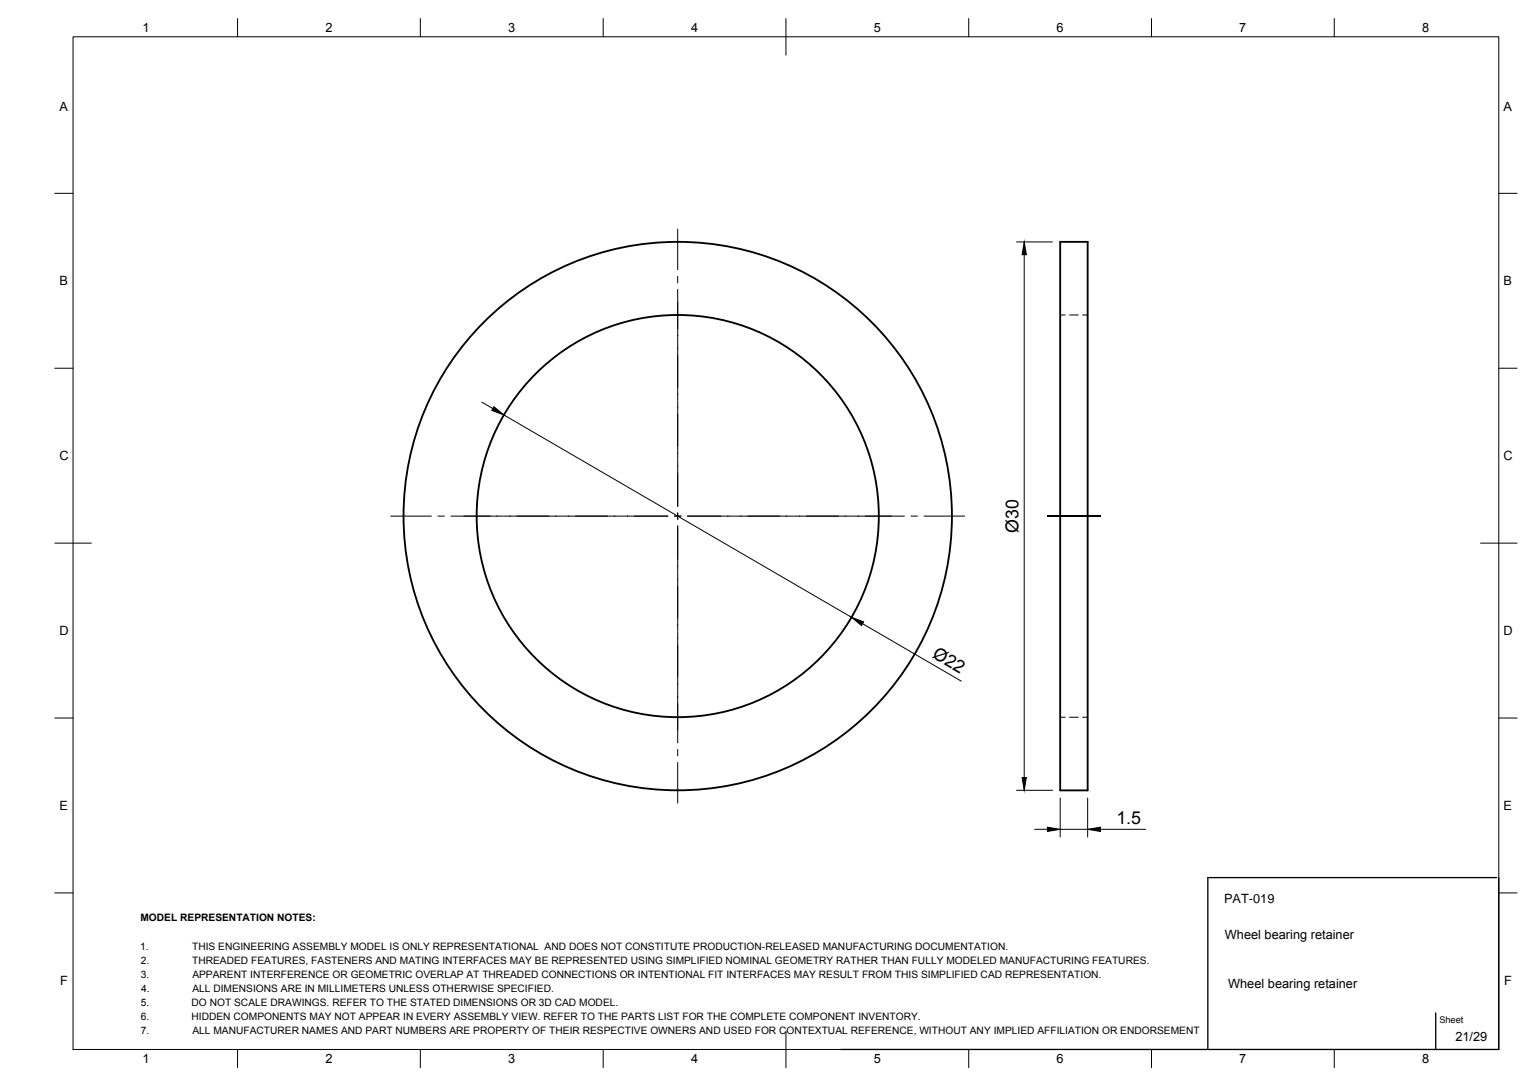
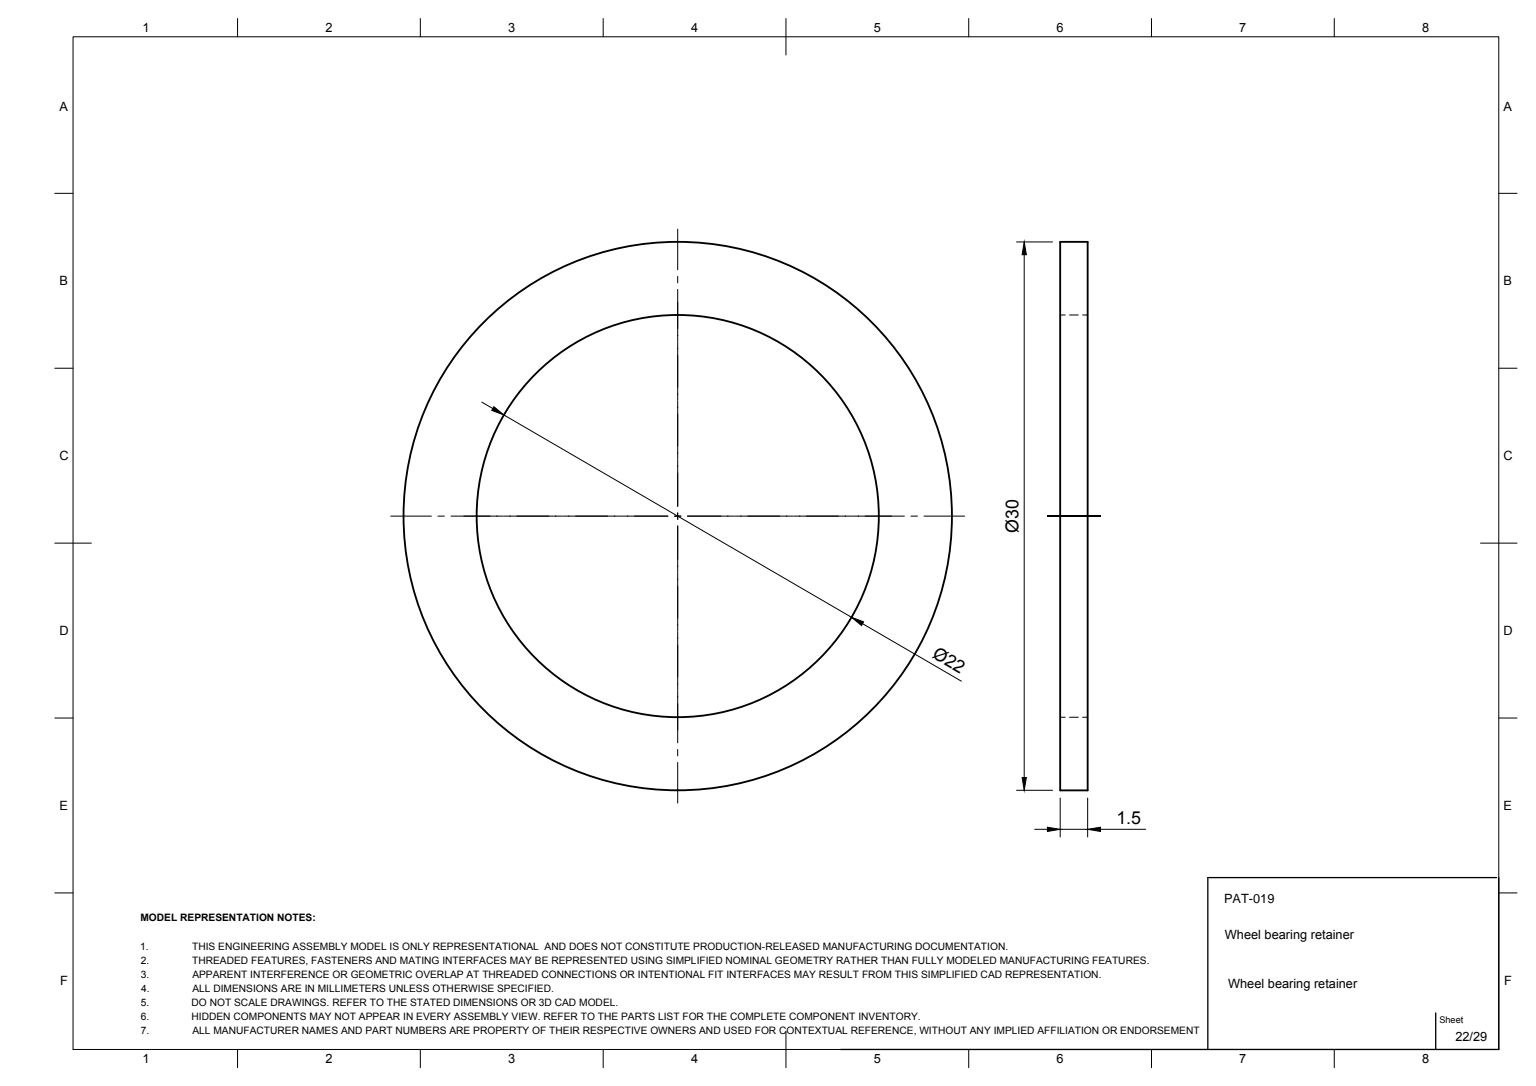
ISO-10303-21;
HEADER;
/* Generated by software containing ST-Developer
 * from STEP Tools, Inc. (www.steptools.com) 
 */

FILE_DESCRIPTION(
/* description */ ('Caster wheel assembly'),
/* implementation_level */ '2;1');

FILE_NAME(
/* name */ 'Wheel bearing retainer.step',
/* time_stamp */ '2026-10-28T03:23:56-07:00',
/* author */ (''),
/* organization */ (''),
/* preprocessor_version */ 'ST-DEVELOPER v20.2',
/* originating_system */ 'Autodesk Translation Framework v15.17.0.0',
/* authorisation */ '');

FILE_SCHEMA (('AUTOMOTIVE_DESIGN { 1 0 10303 214 3 1 1 }'));
ENDSEC;

DATA;
#10=MECHANICAL_DESIGN_GEOMETRIC_PRESENTATION_REPRESENTATION('',(#237),#5385);
#193=SHAPE_REPRESENTATION_RELATIONSHIP('SRR','None',#5490,#215);
#215=ADVANCED_BREP_SHAPE_REPRESENTATION('',(#266),#5377);
#237=STYLED_ITEM('',(#5672),#266);
#266=MANIFOLD_SOLID_BREP('Body1',#2665);
#320=FACE_BOUND('',#740,.T.);
#321=FACE_BOUND('',#742,.T.);
#400=PLANE('',#3151);
#401=PLANE('',#3152);
#530=FACE_OUTER_BOUND('',#737,.T.);
#531=FACE_OUTER_BOUND('',#738,.T.);
#532=FACE_OUTER_BOUND('',#739,.T.);
#533=FACE_OUTER_BOUND('',#741,.T.);
#737=EDGE_LOOP('',(#2192,#2193,#2194,#2195));
#738=EDGE_LOOP('',(#2196,#2197,#2198,#2199));
#739=EDGE_LOOP('',(#2200));
#740=EDGE_LOOP('',(#2201));
#741=EDGE_LOOP('',(#2202));
#742=EDGE_LOOP('',(#2203));
#923=LINE('',#4711,#1057);
#924=LINE('',#4717,#1058);
#1057=VECTOR('',#3866,1.1);
#1058=VECTOR('',#3873,1.5);
#1156=CIRCLE('',#3146,1.1);
#1157=CIRCLE('',#3147,1.1);
#1158=CIRCLE('',#3149,1.5);
#1159=CIRCLE('',#3150,1.5);
#1371=VERTEX_POINT('',#4708);
#1372=VERTEX_POINT('',#4710);
#1373=VERTEX_POINT('',#4714);
#1374=VERTEX_POINT('',#4716);
#1664=EDGE_CURVE('',#1371,#1371,#1156,.T.);
#1665=EDGE_CURVE('',#1371,#1372,#923,.T.);
#1666=EDGE_CURVE('',#1372,#1372,#1157,.T.);
#1667=EDGE_CURVE('',#1373,#1373,#1158,.T.);
#1668=EDGE_CURVE('',#1373,#1374,#924,.T.);
#1669=EDGE_CURVE('',#1374,#1374,#1159,.T.);
#2192=ORIENTED_EDGE('',*,*,#1664,.F.);
#2193=ORIENTED_EDGE('',*,*,#1665,.T.);
#2194=ORIENTED_EDGE('',*,*,#1666,.T.);
#2195=ORIENTED_EDGE('',*,*,#1665,.F.);
#2196=ORIENTED_EDGE('',*,*,#1667,.F.);
#2197=ORIENTED_EDGE('',*,*,#1668,.T.);
#2198=ORIENTED_EDGE('',*,*,#1669,.T.);
#2199=ORIENTED_EDGE('',*,*,#1668,.F.);
#2200=ORIENTED_EDGE('',*,*,#1667,.T.);
#2201=ORIENTED_EDGE('',*,*,#1664,.T.);
#2202=ORIENTED_EDGE('',*,*,#1669,.F.);
#2203=ORIENTED_EDGE('',*,*,#1666,.F.);
#2465=CYLINDRICAL_SURFACE('',#3145,1.1);
#2466=CYLINDRICAL_SURFACE('',#3148,1.5);
#2590=ADVANCED_FACE('',(#530),#2465,.F.);
#2591=ADVANCED_FACE('',(#531),#2466,.T.);
#2592=ADVANCED_FACE('',(#532,#320),#400,.T.);
#2593=ADVANCED_FACE('',(#533,#321),#401,.F.);
#2665=CLOSED_SHELL('',(#2590,#2591,#2592,#2593));
#3144=AXIS2_PLACEMENT_3D('',#4706,#3860,#3861);
#3145=AXIS2_PLACEMENT_3D('',#4707,#3862,#3863);
#3146=AXIS2_PLACEMENT_3D('',#4709,#3864,#3865);
#3147=AXIS2_PLACEMENT_3D('',#4712,#3867,#3868);
#3148=AXIS2_PLACEMENT_3D('',#4713,#3869,#3870);
#3149=AXIS2_PLACEMENT_3D('',#4715,#3871,#3872);
#3150=AXIS2_PLACEMENT_3D('',#4718,#3874,#3875);
#3151=AXIS2_PLACEMENT_3D('',#4719,#3876,#3877);
#3152=AXIS2_PLACEMENT_3D('',#4720,#3878,#3879);
#3860=DIRECTION('axis',(0.,0.,1.));
#3861=DIRECTION('refdir',(1.,0.,0.));
#3862=DIRECTION('center_axis',(0.,1.,0.));
#3863=DIRECTION('ref_axis',(1.,0.,0.));
#3864=DIRECTION('center_axis',(0.,-1.,0.));
#3865=DIRECTION('ref_axis',(1.,0.,0.));
#3866=DIRECTION('',(0.,-1.,0.));
#3867=DIRECTION('center_axis',(0.,-1.,0.));
#3868=DIRECTION('ref_axis',(1.,0.,0.));
#3869=DIRECTION('center_axis',(0.,1.,0.));
#3870=DIRECTION('ref_axis',(1.,0.,0.));
#3871=DIRECTION('center_axis',(0.,1.,0.));
#3872=DIRECTION('ref_axis',(1.,0.,0.));
#3873=DIRECTION('',(0.,-1.,0.));
#3874=DIRECTION('center_axis',(0.,1.,0.));
#3875=DIRECTION('ref_axis',(1.,0.,0.));
#3876=DIRECTION('center_axis',(0.,1.,0.));
#3877=DIRECTION('ref_axis',(1.,0.,0.));
#3878=DIRECTION('center_axis',(0.,1.,0.));
#3879=DIRECTION('ref_axis',(1.,0.,0.));
#4706=CARTESIAN_POINT('',(0.,0.,0.));
#4707=CARTESIAN_POINT('Origin',(0.,-1.2,4.));
#4708=CARTESIAN_POINT('',(-1.1,-1.05,4.));
#4709=CARTESIAN_POINT('Origin',(0.,-1.05,4.));
#4710=CARTESIAN_POINT('',(-1.1,-1.2,4.));
#4711=CARTESIAN_POINT('',(-1.1,-1.2,4.));
#4712=CARTESIAN_POINT('Origin',(0.,-1.2,4.));
#4713=CARTESIAN_POINT('Origin',(0.,-1.2,4.));
#4714=CARTESIAN_POINT('',(-1.5,-1.05,4.));
#4715=CARTESIAN_POINT('Origin',(0.,-1.05,4.));
#4716=CARTESIAN_POINT('',(-1.5,-1.2,4.));
#4717=CARTESIAN_POINT('',(-1.5,-1.2,4.));
#4718=CARTESIAN_POINT('Origin',(0.,-1.2,4.));
#4719=CARTESIAN_POINT('Origin',(0.,-1.05,4.));
#4720=CARTESIAN_POINT('Origin',(0.,-1.2,4.));
#5349=UNCERTAINTY_MEASURE_WITH_UNIT(LENGTH_MEASURE(0.001),#5386,
'DISTANCE_ACCURACY_VALUE',
'Maximum model space distance between geometric entities at asserted c
onnectivities');
#5357=UNCERTAINTY_MEASURE_WITH_UNIT(LENGTH_MEASURE(0.001),#5386,
'DISTANCE_ACCURACY_VALUE',
'Maximum model space distance between geometric entities at asserted c
onnectivities');
#5377=(
GEOMETRIC_REPRESENTATION_CONTEXT(3)
GLOBAL_UNCERTAINTY_ASSIGNED_CONTEXT((#5349))
GLOBAL_UNIT_ASSIGNED_CONTEXT((#5386,#5388,#5389))
REPRESENTATION_CONTEXT('','3D')
);
#5385=(
GEOMETRIC_REPRESENTATION_CONTEXT(3)
GLOBAL_UNCERTAINTY_ASSIGNED_CONTEXT((#5357))
GLOBAL_UNIT_ASSIGNED_CONTEXT((#5386,#5388,#5389))
REPRESENTATION_CONTEXT('','3D')
);
#5386=(
LENGTH_UNIT()
NAMED_UNIT(*)
SI_UNIT(.CENTI.,.METRE.)
);
#5388=(
NAMED_UNIT(*)
PLANE_ANGLE_UNIT()
SI_UNIT($,.RADIAN.)
);
#5389=(
NAMED_UNIT(*)
SI_UNIT($,.STERADIAN.)
SOLID_ANGLE_UNIT()
);
#5409=SHAPE_DEFINITION_REPRESENTATION(#5450,#5490);
#5450=PRODUCT_DEFINITION_SHAPE('',$,#5518);
#5490=SHAPE_REPRESENTATION('',(#3144),#5377);
#5498=PRODUCT_DEFINITION_CONTEXT('part definition',#5581,'design');
#5518=PRODUCT_DEFINITION('Wheel bearing retainer',
'Wheel bearing retainer',#5545,#5498);
#5545=PRODUCT_DEFINITION_FORMATION('',$,#5602);
#5581=APPLICATION_CONTEXT(
'Core Data for Automotive Mechanical Design Process');
#5582=PRODUCT_CONTEXT('part definition',#5581,'mechanical');
#5602=PRODUCT('Wheel bearing retainer','Wheel bearing retainer',
'Wheel bearing retainer',(#5582));
#5666=COLOUR_RGB('Grey',0.48,0.52,0.57);
#5667=FILL_AREA_STYLE_COLOUR('',#5666);
#5668=FILL_AREA_STYLE('',(#5667));
#5669=SURFACE_STYLE_FILL_AREA(#5668);
#5670=SURFACE_SIDE_STYLE('',(#5669));
#5671=SURFACE_STYLE_USAGE(.BOTH.,#5670);
#5672=PRESENTATION_STYLE_ASSIGNMENT((#5671));
ENDSEC;
END-ISO-10303-21;
